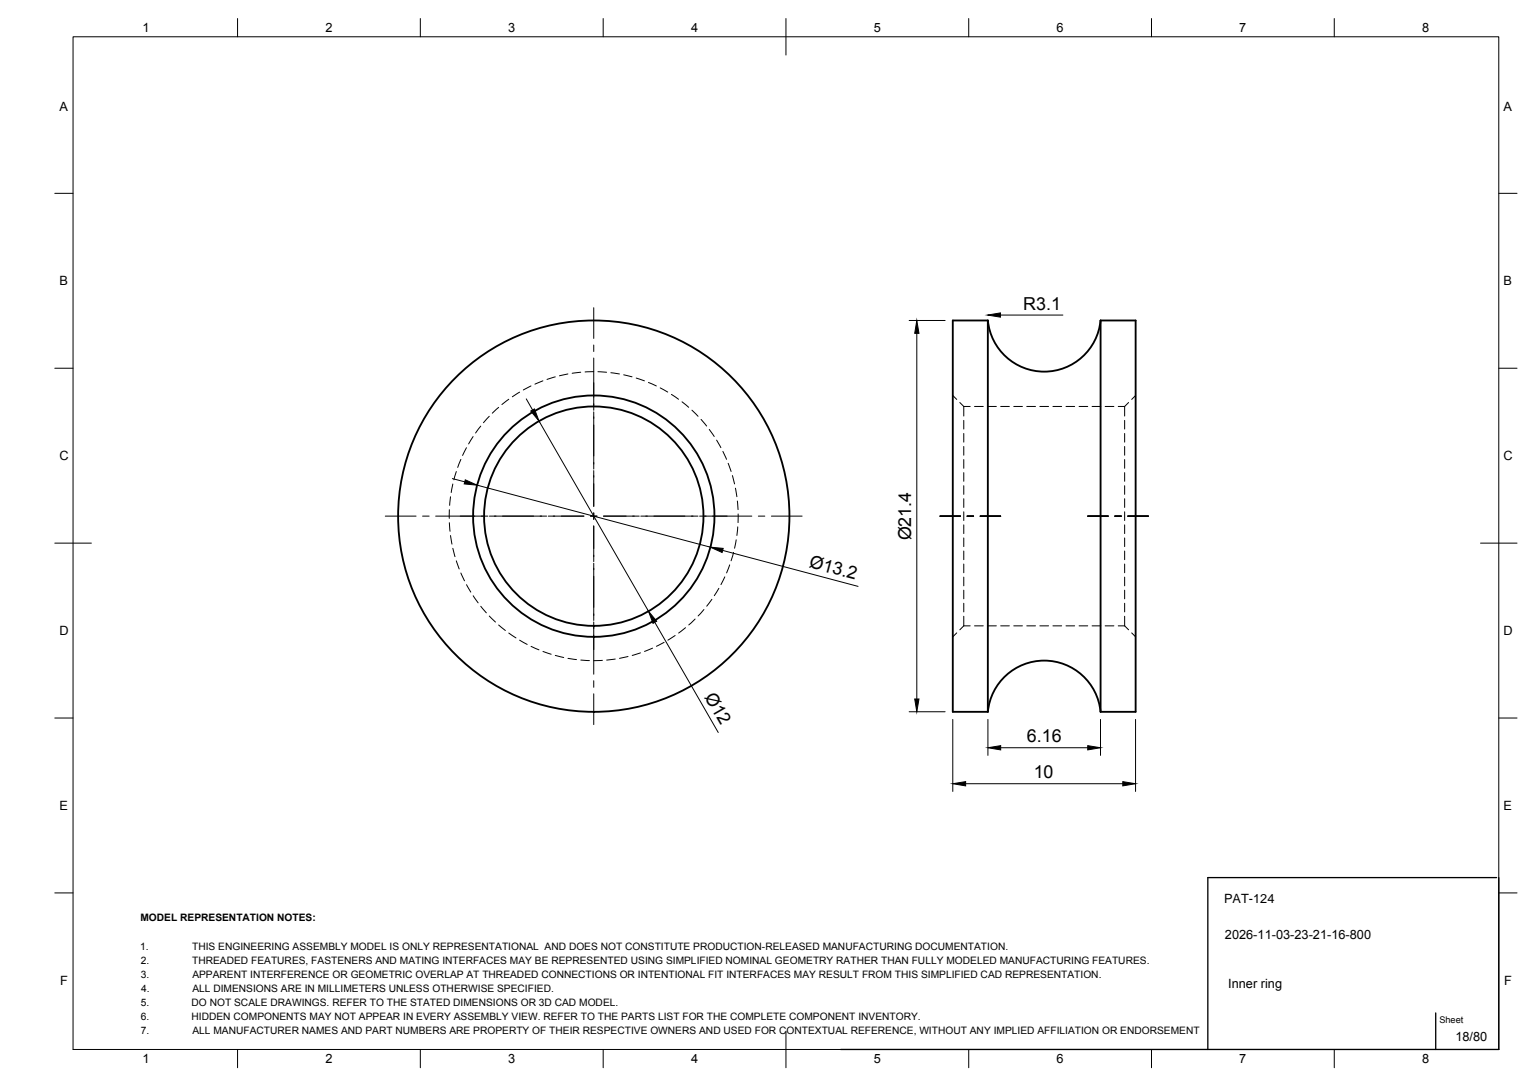
ISO-10303-21;
HEADER;
/* Generated by software containing ST-Developer
 * from STEP Tools, Inc. (www.steptools.com) 
 */

FILE_DESCRIPTION(
/* description */ ('XY cross-slide table'),
/* implementation_level */ '2;1');

FILE_NAME(
/* name */ 'Inner ring.step',
/* time_stamp */ '2026-10-28T03:22:46-07:00',
/* author */ (''),
/* organization */ (''),
/* preprocessor_version */ 'ST-DEVELOPER v20.2',
/* originating_system */ 'Autodesk Translation Framework v15.17.0.0',
/* authorisation */ '');

FILE_SCHEMA (('AUTOMOTIVE_DESIGN { 1 0 10303 214 3 1 1 }'));
ENDSEC;

DATA;
#10=MECHANICAL_DESIGN_GEOMETRIC_PRESENTATION_REPRESENTATION('',(#1681),#62984);
#1441=CONICAL_SURFACE('',#24298,0.63,0.785398163397448);
#1442=CONICAL_SURFACE('',#24305,0.63,0.785398163397448);
#1496=TOROIDAL_SURFACE('',#24287,1.1,0.309556);
#1515=SHAPE_REPRESENTATION_RELATIONSHIP('SRR','None',#63364,#1598);
#1598=ADVANCED_BREP_SHAPE_REPRESENTATION('',(#1794),#62901);
#1681=STYLED_ITEM('',(#63912),#1794);
#1794=MANIFOLD_SOLID_BREP('Body1',#22975);
#1983=FACE_BOUND('',#4431,.T.);
#1984=FACE_BOUND('',#4434,.T.);
#2381=PLANE('',#24300);
#2382=PLANE('',#24303);
#3016=FACE_OUTER_BOUND('',#4426,.T.);
#3017=FACE_OUTER_BOUND('',#4427,.T.);
#3018=FACE_OUTER_BOUND('',#4428,.T.);
#3019=FACE_OUTER_BOUND('',#4429,.T.);
#3020=FACE_OUTER_BOUND('',#4430,.T.);
#3021=FACE_OUTER_BOUND('',#4432,.T.);
#3022=FACE_OUTER_BOUND('',#4433,.T.);
#3023=FACE_OUTER_BOUND('',#4435,.T.);
#4426=EDGE_LOOP('',(#15554,#15555,#15556,#15557,#15558,#15559));
#4427=EDGE_LOOP('',(#15560,#15561,#15562,#15563,#15564));
#4428=EDGE_LOOP('',(#15565,#15566,#15567,#15568));
#4429=EDGE_LOOP('',(#15569,#15570,#15571,#15572));
#4430=EDGE_LOOP('',(#15573));
#4431=EDGE_LOOP('',(#15574));
#4432=EDGE_LOOP('',(#15575,#15576,#15577,#15578,#15579));
#4433=EDGE_LOOP('',(#15580));
#4434=EDGE_LOOP('',(#15581));
#4435=EDGE_LOOP('',(#15582,#15583,#15584,#15585));
#6107=LINE('',#33584,#7594);
#6108=LINE('',#33590,#7595);
#6109=LINE('',#33594,#7596);
#6110=LINE('',#33600,#7597);
#6111=LINE('',#33605,#7598);
#7594=VECTOR('',#27250,1.070235);
#7595=VECTOR('',#27257,0.6);
#7596=VECTOR('',#27262,0.63);
#7597=VECTOR('',#27271,1.070235);
#7598=VECTOR('',#27278,0.63);
#9004=CIRCLE('',#24288,1.070235);
#9005=CIRCLE('',#24289,1.070235);
#9006=CIRCLE('',#24290,0.309556);
#9007=CIRCLE('',#24291,1.070235);
#9008=CIRCLE('',#24292,1.070235);
#9009=CIRCLE('',#24294,1.070235);
#9010=CIRCLE('',#24296,0.6);
#9011=CIRCLE('',#24297,0.6);
#9012=CIRCLE('',#24299,0.66);
#9013=CIRCLE('',#24302,1.070235);
#9014=CIRCLE('',#24304,0.66);
#9987=VERTEX_POINT('',#33573);
#9988=VERTEX_POINT('',#33574);
#9989=VERTEX_POINT('',#33577);
#9990=VERTEX_POINT('',#33579);
#9991=VERTEX_POINT('',#33583);
#9992=VERTEX_POINT('',#33587);
#9993=VERTEX_POINT('',#33589);
#9994=VERTEX_POINT('',#33593);
#9995=VERTEX_POINT('',#33598);
#9996=VERTEX_POINT('',#33602);
#12161=EDGE_CURVE('',#9987,#9988,#9004,.T.);
#12162=EDGE_CURVE('',#9988,#9987,#9005,.T.);
#12163=EDGE_CURVE('',#9988,#9989,#9006,.T.);
#12164=EDGE_CURVE('',#9990,#9989,#9007,.T.);
#12165=EDGE_CURVE('',#9989,#9990,#9008,.T.);
#12166=EDGE_CURVE('',#9990,#9991,#6107,.T.);
#12167=EDGE_CURVE('',#9991,#9991,#9009,.T.);
#12168=EDGE_CURVE('',#9992,#9992,#9010,.T.);
#12169=EDGE_CURVE('',#9992,#9993,#6108,.T.);
#12170=EDGE_CURVE('',#9993,#9993,#9011,.T.);
#12171=EDGE_CURVE('',#9993,#9994,#6109,.T.);
#12172=EDGE_CURVE('',#9994,#9994,#9012,.T.);
#12173=EDGE_CURVE('',#9995,#9995,#9013,.T.);
#12174=EDGE_CURVE('',#9995,#9987,#6110,.T.);
#12175=EDGE_CURVE('',#9996,#9996,#9014,.T.);
#12176=EDGE_CURVE('',#9996,#9992,#6111,.T.);
#15554=ORIENTED_EDGE('',*,*,#12161,.F.);
#15555=ORIENTED_EDGE('',*,*,#12162,.F.);
#15556=ORIENTED_EDGE('',*,*,#12163,.T.);
#15557=ORIENTED_EDGE('',*,*,#12164,.F.);
#15558=ORIENTED_EDGE('',*,*,#12165,.F.);
#15559=ORIENTED_EDGE('',*,*,#12163,.F.);
#15560=ORIENTED_EDGE('',*,*,#12164,.T.);
#15561=ORIENTED_EDGE('',*,*,#12165,.T.);
#15562=ORIENTED_EDGE('',*,*,#12166,.T.);
#15563=ORIENTED_EDGE('',*,*,#12167,.T.);
#15564=ORIENTED_EDGE('',*,*,#12166,.F.);
#15565=ORIENTED_EDGE('',*,*,#12168,.T.);
#15566=ORIENTED_EDGE('',*,*,#12169,.T.);
#15567=ORIENTED_EDGE('',*,*,#12170,.F.);
#15568=ORIENTED_EDGE('',*,*,#12169,.F.);
#15569=ORIENTED_EDGE('',*,*,#12170,.T.);
#15570=ORIENTED_EDGE('',*,*,#12171,.T.);
#15571=ORIENTED_EDGE('',*,*,#12172,.F.);
#15572=ORIENTED_EDGE('',*,*,#12171,.F.);
#15573=ORIENTED_EDGE('',*,*,#12167,.F.);
#15574=ORIENTED_EDGE('',*,*,#12172,.T.);
#15575=ORIENTED_EDGE('',*,*,#12173,.F.);
#15576=ORIENTED_EDGE('',*,*,#12174,.T.);
#15577=ORIENTED_EDGE('',*,*,#12161,.T.);
#15578=ORIENTED_EDGE('',*,*,#12162,.T.);
#15579=ORIENTED_EDGE('',*,*,#12174,.F.);
#15580=ORIENTED_EDGE('',*,*,#12173,.T.);
#15581=ORIENTED_EDGE('',*,*,#12175,.F.);
#15582=ORIENTED_EDGE('',*,*,#12175,.T.);
#15583=ORIENTED_EDGE('',*,*,#12176,.T.);
#15584=ORIENTED_EDGE('',*,*,#12168,.F.);
#15585=ORIENTED_EDGE('',*,*,#12176,.F.);
#21102=CYLINDRICAL_SURFACE('',#24293,1.070235);
#21103=CYLINDRICAL_SURFACE('',#24295,0.6);
#21104=CYLINDRICAL_SURFACE('',#24301,1.070235);
#21797=ADVANCED_FACE('',(#3016),#1496,.F.);
#21798=ADVANCED_FACE('',(#3017),#21102,.T.);
#21799=ADVANCED_FACE('',(#3018),#21103,.F.);
#21800=ADVANCED_FACE('',(#3019),#1441,.F.);
#21801=ADVANCED_FACE('',(#3020,#1983),#2381,.T.);
#21802=ADVANCED_FACE('',(#3021),#21104,.T.);
#21803=ADVANCED_FACE('',(#3022,#1984),#2382,.T.);
#21804=ADVANCED_FACE('',(#3023),#1442,.F.);
#22975=CLOSED_SHELL('',(#21797,#21798,#21799,#21800,#21801,#21802,#21803,
#21804));
#24286=AXIS2_PLACEMENT_3D('',#33571,#27234,#27235);
#24287=AXIS2_PLACEMENT_3D('',#33572,#27236,#27237);
#24288=AXIS2_PLACEMENT_3D('',#33575,#27238,#27239);
#24289=AXIS2_PLACEMENT_3D('',#33576,#27240,#27241);
#24290=AXIS2_PLACEMENT_3D('',#33578,#27242,#27243);
#24291=AXIS2_PLACEMENT_3D('',#33580,#27244,#27245);
#24292=AXIS2_PLACEMENT_3D('',#33581,#27246,#27247);
#24293=AXIS2_PLACEMENT_3D('',#33582,#27248,#27249);
#24294=AXIS2_PLACEMENT_3D('',#33585,#27251,#27252);
#24295=AXIS2_PLACEMENT_3D('',#33586,#27253,#27254);
#24296=AXIS2_PLACEMENT_3D('',#33588,#27255,#27256);
#24297=AXIS2_PLACEMENT_3D('',#33591,#27258,#27259);
#24298=AXIS2_PLACEMENT_3D('',#33592,#27260,#27261);
#24299=AXIS2_PLACEMENT_3D('',#33595,#27263,#27264);
#24300=AXIS2_PLACEMENT_3D('',#33596,#27265,#27266);
#24301=AXIS2_PLACEMENT_3D('',#33597,#27267,#27268);
#24302=AXIS2_PLACEMENT_3D('',#33599,#27269,#27270);
#24303=AXIS2_PLACEMENT_3D('',#33601,#27272,#27273);
#24304=AXIS2_PLACEMENT_3D('',#33603,#27274,#27275);
#24305=AXIS2_PLACEMENT_3D('',#33604,#27276,#27277);
#27234=DIRECTION('axis',(0.,0.,1.));
#27235=DIRECTION('refdir',(1.,0.,0.));
#27236=DIRECTION('center_axis',(0.,-1.,0.));
#27237=DIRECTION('ref_axis',(0.,0.,-1.));
#27238=DIRECTION('center_axis',(0.,-1.,0.));
#27239=DIRECTION('ref_axis',(1.,0.,0.));
#27240=DIRECTION('center_axis',(0.,-1.,0.));
#27241=DIRECTION('ref_axis',(1.,0.,0.));
#27242=DIRECTION('center_axis',(1.,0.,1.22464679914735E-16));
#27243=DIRECTION('ref_axis',(-1.22464679914735E-16,0.,1.));
#27244=DIRECTION('center_axis',(0.,1.,0.));
#27245=DIRECTION('ref_axis',(1.,0.,0.));
#27246=DIRECTION('center_axis',(0.,1.,0.));
#27247=DIRECTION('ref_axis',(1.,0.,0.));
#27248=DIRECTION('center_axis',(0.,-1.,0.));
#27249=DIRECTION('ref_axis',(1.,0.,0.));
#27250=DIRECTION('',(0.,1.,0.));
#27251=DIRECTION('center_axis',(0.,-1.,0.));
#27252=DIRECTION('ref_axis',(1.,0.,0.));
#27253=DIRECTION('center_axis',(0.,-1.,0.));
#27254=DIRECTION('ref_axis',(1.,0.,0.));
#27255=DIRECTION('center_axis',(0.,-1.,0.));
#27256=DIRECTION('ref_axis',(1.,0.,0.));
#27257=DIRECTION('',(0.,1.,0.));
#27258=DIRECTION('center_axis',(0.,-1.,0.));
#27259=DIRECTION('ref_axis',(1.,0.,0.));
#27260=DIRECTION('center_axis',(0.,1.,0.));
#27261=DIRECTION('ref_axis',(1.,0.,0.));
#27262=DIRECTION('',(-0.707106781186548,0.707106781186547,-8.65956056235493E-17));
#27263=DIRECTION('center_axis',(0.,-1.,0.));
#27264=DIRECTION('ref_axis',(1.,0.,0.));
#27265=DIRECTION('center_axis',(0.,1.,0.));
#27266=DIRECTION('ref_axis',(0.,0.,1.));
#27267=DIRECTION('center_axis',(0.,-1.,0.));
#27268=DIRECTION('ref_axis',(1.,0.,0.));
#27269=DIRECTION('center_axis',(0.,-1.,0.));
#27270=DIRECTION('ref_axis',(1.,0.,0.));
#27271=DIRECTION('',(0.,1.,0.));
#27272=DIRECTION('center_axis',(0.,-1.,0.));
#27273=DIRECTION('ref_axis',(0.,0.,-1.));
#27274=DIRECTION('center_axis',(0.,-1.,0.));
#27275=DIRECTION('ref_axis',(1.,0.,0.));
#27276=DIRECTION('center_axis',(0.,-1.,0.));
#27277=DIRECTION('ref_axis',(1.,0.,0.));
#27278=DIRECTION('',(0.707106781186548,0.707106781186547,8.65956056235493E-17));
#33571=CARTESIAN_POINT('',(0.,0.,0.));
#33572=CARTESIAN_POINT('Origin',(0.,0.,0.));
#33573=CARTESIAN_POINT('',(-1.070235,-0.308121667383195,-1.31065986708547E-16));
#33574=CARTESIAN_POINT('',(-1.31065986708547E-16,-0.308121667383195,1.070235));
#33575=CARTESIAN_POINT('Origin',(0.,-0.308121667383195,0.));
#33576=CARTESIAN_POINT('Origin',(0.,-0.308121667383195,0.));
#33577=CARTESIAN_POINT('',(-1.31065986708547E-16,0.308121667383195,1.070235));
#33578=CARTESIAN_POINT('Origin',(-1.34711147906209E-16,0.,1.1));
#33579=CARTESIAN_POINT('',(-1.070235,0.308121667383195,1.31065986708547E-16));
#33580=CARTESIAN_POINT('Origin',(0.,0.308121667383195,0.));
#33581=CARTESIAN_POINT('Origin',(0.,0.308121667383195,0.));
#33582=CARTESIAN_POINT('Origin',(0.,0.,0.));
#33583=CARTESIAN_POINT('',(-1.070235,0.5,-1.31065986708547E-16));
#33584=CARTESIAN_POINT('',(-1.070235,0.,-1.31065986708547E-16));
#33585=CARTESIAN_POINT('Origin',(0.,0.5,0.));
#33586=CARTESIAN_POINT('Origin',(0.,0.,0.));
#33587=CARTESIAN_POINT('',(-0.6,-0.44,-7.34788079488412E-17));
#33588=CARTESIAN_POINT('Origin',(0.,-0.44,0.));
#33589=CARTESIAN_POINT('',(-0.6,0.44,-7.34788079488412E-17));
#33590=CARTESIAN_POINT('',(-0.6,0.,-7.34788079488412E-17));
#33591=CARTESIAN_POINT('Origin',(0.,0.44,0.));
#33592=CARTESIAN_POINT('Origin',(0.,0.47,0.));
#33593=CARTESIAN_POINT('',(-0.66,0.5,-8.08266887437253E-17));
#33594=CARTESIAN_POINT('',(-0.63,0.47,-7.71527483462832E-17));
#33595=CARTESIAN_POINT('Origin',(0.,0.5,0.));
#33596=CARTESIAN_POINT('Origin',(1.070235,0.5,0.));
#33597=CARTESIAN_POINT('Origin',(0.,0.,0.));
#33598=CARTESIAN_POINT('',(-1.070235,-0.5,-1.31065986708547E-16));
#33599=CARTESIAN_POINT('Origin',(0.,-0.5,0.));
#33600=CARTESIAN_POINT('',(-1.070235,0.,-1.31065986708547E-16));
#33601=CARTESIAN_POINT('Origin',(0.66,-0.5,0.));
#33602=CARTESIAN_POINT('',(-0.66,-0.5,-8.08266887437253E-17));
#33603=CARTESIAN_POINT('Origin',(0.,-0.5,0.));
#33604=CARTESIAN_POINT('Origin',(0.,-0.47,0.));
#33605=CARTESIAN_POINT('',(-0.63,-0.47,-7.71527483462832E-17));
#62802=UNCERTAINTY_MEASURE_WITH_UNIT(LENGTH_MEASURE(0.001),#62985,
'DISTANCE_ACCURACY_VALUE',
'Maximum model space distance between geometric entities at asserted c
onnectivities');
#62885=UNCERTAINTY_MEASURE_WITH_UNIT(LENGTH_MEASURE(0.001),#62985,
'DISTANCE_ACCURACY_VALUE',
'Maximum model space distance between geometric entities at asserted c
onnectivities');
#62901=(
GEOMETRIC_REPRESENTATION_CONTEXT(3)
GLOBAL_UNCERTAINTY_ASSIGNED_CONTEXT((#62802))
GLOBAL_UNIT_ASSIGNED_CONTEXT((#62985,#62987,#62988))
REPRESENTATION_CONTEXT('','3D')
);
#62984=(
GEOMETRIC_REPRESENTATION_CONTEXT(3)
GLOBAL_UNCERTAINTY_ASSIGNED_CONTEXT((#62885))
GLOBAL_UNIT_ASSIGNED_CONTEXT((#62985,#62987,#62988))
REPRESENTATION_CONTEXT('','3D')
);
#62985=(
LENGTH_UNIT()
NAMED_UNIT(*)
SI_UNIT(.CENTI.,.METRE.)
);
#62987=(
NAMED_UNIT(*)
PLANE_ANGLE_UNIT()
SI_UNIT($,.RADIAN.)
);
#62988=(
NAMED_UNIT(*)
SI_UNIT($,.STERADIAN.)
SOLID_ANGLE_UNIT()
);
#63004=SHAPE_DEFINITION_REPRESENTATION(#63102,#63364);
#63102=PRODUCT_DEFINITION_SHAPE('',$,#63463);
#63364=SHAPE_REPRESENTATION('',(#24286),#62901);
#63447=PRODUCT_DEFINITION_CONTEXT('part definition',#63743,'design');
#63463=PRODUCT_DEFINITION('Inner ring','Inner ring',#63561,#63447);
#63561=PRODUCT_DEFINITION_FORMATION('',$,#63760);
#63743=APPLICATION_CONTEXT(
'Core Data for Automotive Mechanical Design Process');
#63744=PRODUCT_CONTEXT('part definition',#63743,'mechanical');
#63760=PRODUCT('Inner ring','Inner ring','Inner ring',(#63744));
#63906=COLOUR_RGB('Grey',0.48,0.52,0.57);
#63907=FILL_AREA_STYLE_COLOUR('',#63906);
#63908=FILL_AREA_STYLE('',(#63907));
#63909=SURFACE_STYLE_FILL_AREA(#63908);
#63910=SURFACE_SIDE_STYLE('',(#63909));
#63911=SURFACE_STYLE_USAGE(.BOTH.,#63910);
#63912=PRESENTATION_STYLE_ASSIGNMENT((#63911));
ENDSEC;
END-ISO-10303-21;
